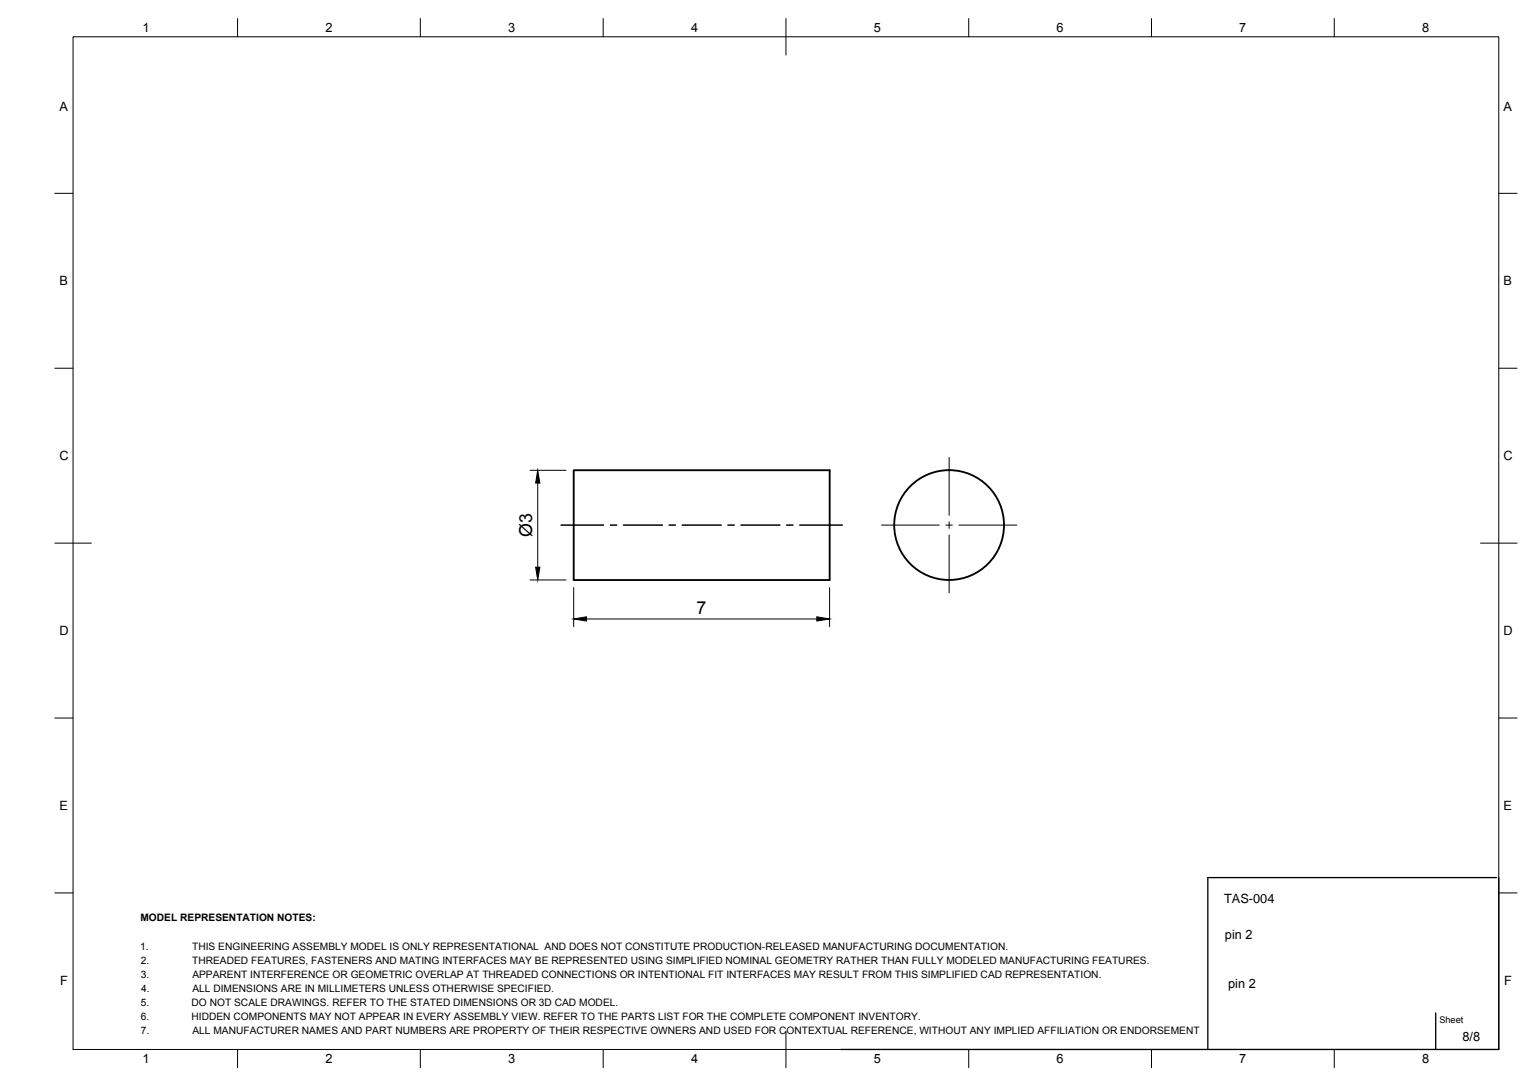
ISO-10303-21;
HEADER;
/* Generated by software containing ST-Developer
 * from STEP Tools, Inc. (www.steptools.com) 
 */

FILE_DESCRIPTION(
/* description */ ('STEP AP214'),
/* implementation_level */ '2;1');

FILE_NAME(
/* name */ 'pin 2.step',
/* time_stamp */ '2026-11-04T19:48:07-08:00',
/* author */ (''),
/* organization */ (''),
/* preprocessor_version */ 'ST-DEVELOPER v20.2',
/* originating_system */ 'Autodesk Translation Framework v15.17.0.0',
/* authorisation */ '');

FILE_SCHEMA (('AUTOMOTIVE_DESIGN { 1 0 10303 214 3 1 1 }'));
ENDSEC;

DATA;
#10=MECHANICAL_DESIGN_GEOMETRIC_PRESENTATION_REPRESENTATION('',(#64),#9561);
#52=SHAPE_REPRESENTATION_RELATIONSHIP('SRR','None',#9592,#58);
#58=ADVANCED_BREP_SHAPE_REPRESENTATION('',(#70),#9560);
#64=STYLED_ITEM('',(#9629),#70);
#70=MANIFOLD_SOLID_BREP('Body1',#2410);
#192=PLANE('',#2688);
#193=PLANE('',#2689);
#334=FACE_OUTER_BOUND('',#492,.T.);
#335=FACE_OUTER_BOUND('',#493,.T.);
#336=FACE_OUTER_BOUND('',#494,.T.);
#492=EDGE_LOOP('',(#2225,#2226,#2227,#2228));
#493=EDGE_LOOP('',(#2229));
#494=EDGE_LOOP('',(#2230));
#744=LINE('',#9536,#994);
#994=VECTOR('',#3363,1.5);
#1059=CIRCLE('',#2686,1.5);
#1060=CIRCLE('',#2687,1.5);
#1257=VERTEX_POINT('',#9533);
#1258=VERTEX_POINT('',#9535);
#1580=EDGE_CURVE('',#1257,#1257,#1059,.T.);
#1581=EDGE_CURVE('',#1257,#1258,#744,.T.);
#1582=EDGE_CURVE('',#1258,#1258,#1060,.T.);
#2225=ORIENTED_EDGE('',*,*,#1580,.T.);
#2226=ORIENTED_EDGE('',*,*,#1581,.T.);
#2227=ORIENTED_EDGE('',*,*,#1582,.F.);
#2228=ORIENTED_EDGE('',*,*,#1581,.F.);
#2229=ORIENTED_EDGE('',*,*,#1582,.T.);
#2230=ORIENTED_EDGE('',*,*,#1580,.F.);
#2261=CYLINDRICAL_SURFACE('',#2685,1.5);
#2402=ADVANCED_FACE('',(#334),#2261,.T.);
#2403=ADVANCED_FACE('',(#335),#192,.T.);
#2404=ADVANCED_FACE('',(#336),#193,.F.);
#2410=CLOSED_SHELL('',(#2402,#2403,#2404));
#2684=AXIS2_PLACEMENT_3D('',#9531,#3357,#3358);
#2685=AXIS2_PLACEMENT_3D('',#9532,#3359,#3360);
#2686=AXIS2_PLACEMENT_3D('',#9534,#3361,#3362);
#2687=AXIS2_PLACEMENT_3D('',#9537,#3364,#3365);
#2688=AXIS2_PLACEMENT_3D('',#9538,#3366,#3367);
#2689=AXIS2_PLACEMENT_3D('',#9539,#3368,#3369);
#3357=DIRECTION('axis',(0.,0.,1.));
#3358=DIRECTION('refdir',(1.,0.,0.));
#3359=DIRECTION('center_axis',(0.,0.,-1.));
#3360=DIRECTION('ref_axis',(-1.,0.,0.));
#3361=DIRECTION('center_axis',(0.,0.,1.));
#3362=DIRECTION('ref_axis',(1.,0.,0.));
#3363=DIRECTION('',(0.,0.,1.));
#3364=DIRECTION('center_axis',(0.,0.,1.));
#3365=DIRECTION('ref_axis',(1.,0.,0.));
#3366=DIRECTION('center_axis',(0.,0.,1.));
#3367=DIRECTION('ref_axis',(1.,0.,0.));
#3368=DIRECTION('center_axis',(0.,0.,1.));
#3369=DIRECTION('ref_axis',(1.,0.,0.));
#9531=CARTESIAN_POINT('',(0.,0.,0.));
#9532=CARTESIAN_POINT('Origin',(0.,-10.,3.5));
#9533=CARTESIAN_POINT('',(1.5,-10.,-3.5));
#9534=CARTESIAN_POINT('Origin',(0.,-10.,-3.5));
#9535=CARTESIAN_POINT('',(1.5,-10.,3.5));
#9536=CARTESIAN_POINT('',(1.5,-10.,3.5));
#9537=CARTESIAN_POINT('Origin',(0.,-10.,3.5));
#9538=CARTESIAN_POINT('Origin',(0.,-10.,3.5));
#9539=CARTESIAN_POINT('Origin',(0.,-10.,-3.5));
#9552=UNCERTAINTY_MEASURE_WITH_UNIT(LENGTH_MEASURE(0.01),#9562,
'DISTANCE_ACCURACY_VALUE',
'Maximum model space distance between geometric entities at asserted c
onnectivities');
#9553=UNCERTAINTY_MEASURE_WITH_UNIT(LENGTH_MEASURE(0.01),#9562,
'DISTANCE_ACCURACY_VALUE',
'Maximum model space distance between geometric entities at asserted c
onnectivities');
#9560=(
GEOMETRIC_REPRESENTATION_CONTEXT(3)
GLOBAL_UNCERTAINTY_ASSIGNED_CONTEXT((#9552))
GLOBAL_UNIT_ASSIGNED_CONTEXT((#9562,#9564,#9565))
REPRESENTATION_CONTEXT('','3D')
);
#9561=(
GEOMETRIC_REPRESENTATION_CONTEXT(3)
GLOBAL_UNCERTAINTY_ASSIGNED_CONTEXT((#9553))
GLOBAL_UNIT_ASSIGNED_CONTEXT((#9562,#9564,#9565))
REPRESENTATION_CONTEXT('','3D')
);
#9562=(
LENGTH_UNIT()
NAMED_UNIT(*)
SI_UNIT(.MILLI.,.METRE.)
);
#9564=(
NAMED_UNIT(*)
PLANE_ANGLE_UNIT()
SI_UNIT($,.RADIAN.)
);
#9565=(
NAMED_UNIT(*)
SI_UNIT($,.STERADIAN.)
SOLID_ANGLE_UNIT()
);
#9572=SHAPE_DEFINITION_REPRESENTATION(#9579,#9592);
#9579=PRODUCT_DEFINITION_SHAPE('',$,#9600);
#9592=SHAPE_REPRESENTATION('',(#2684),#9560);
#9593=PRODUCT_DEFINITION_CONTEXT('part definition',#9616,'design');
#9600=PRODUCT_DEFINITION('pin 2','pin 2',#9607,#9593);
#9607=PRODUCT_DEFINITION_FORMATION('',$,#9624);
#9616=APPLICATION_CONTEXT(
'Core Data for Automotive Mechanical Design Process');
#9617=PRODUCT_CONTEXT('part definition',#9616,'mechanical');
#9624=PRODUCT('pin 2','pin 2',$,(#9617));
#9629=PRESENTATION_STYLE_ASSIGNMENT((#9634));
#9634=SURFACE_STYLE_USAGE(.BOTH.,#9639);
#9639=SURFACE_SIDE_STYLE('',(#9644));
#9644=SURFACE_STYLE_FILL_AREA(#9649);
#9649=FILL_AREA_STYLE('Opaque(122,133,145)',(#9654));
#9654=FILL_AREA_STYLE_COLOUR('Opaque(122,133,145)',#9659);
#9659=COLOUR_RGB('Opaque(122,133,145)',0.47843137254902,0.52156862745098,
0.568627450980392);
ENDSEC;
END-ISO-10303-21;
